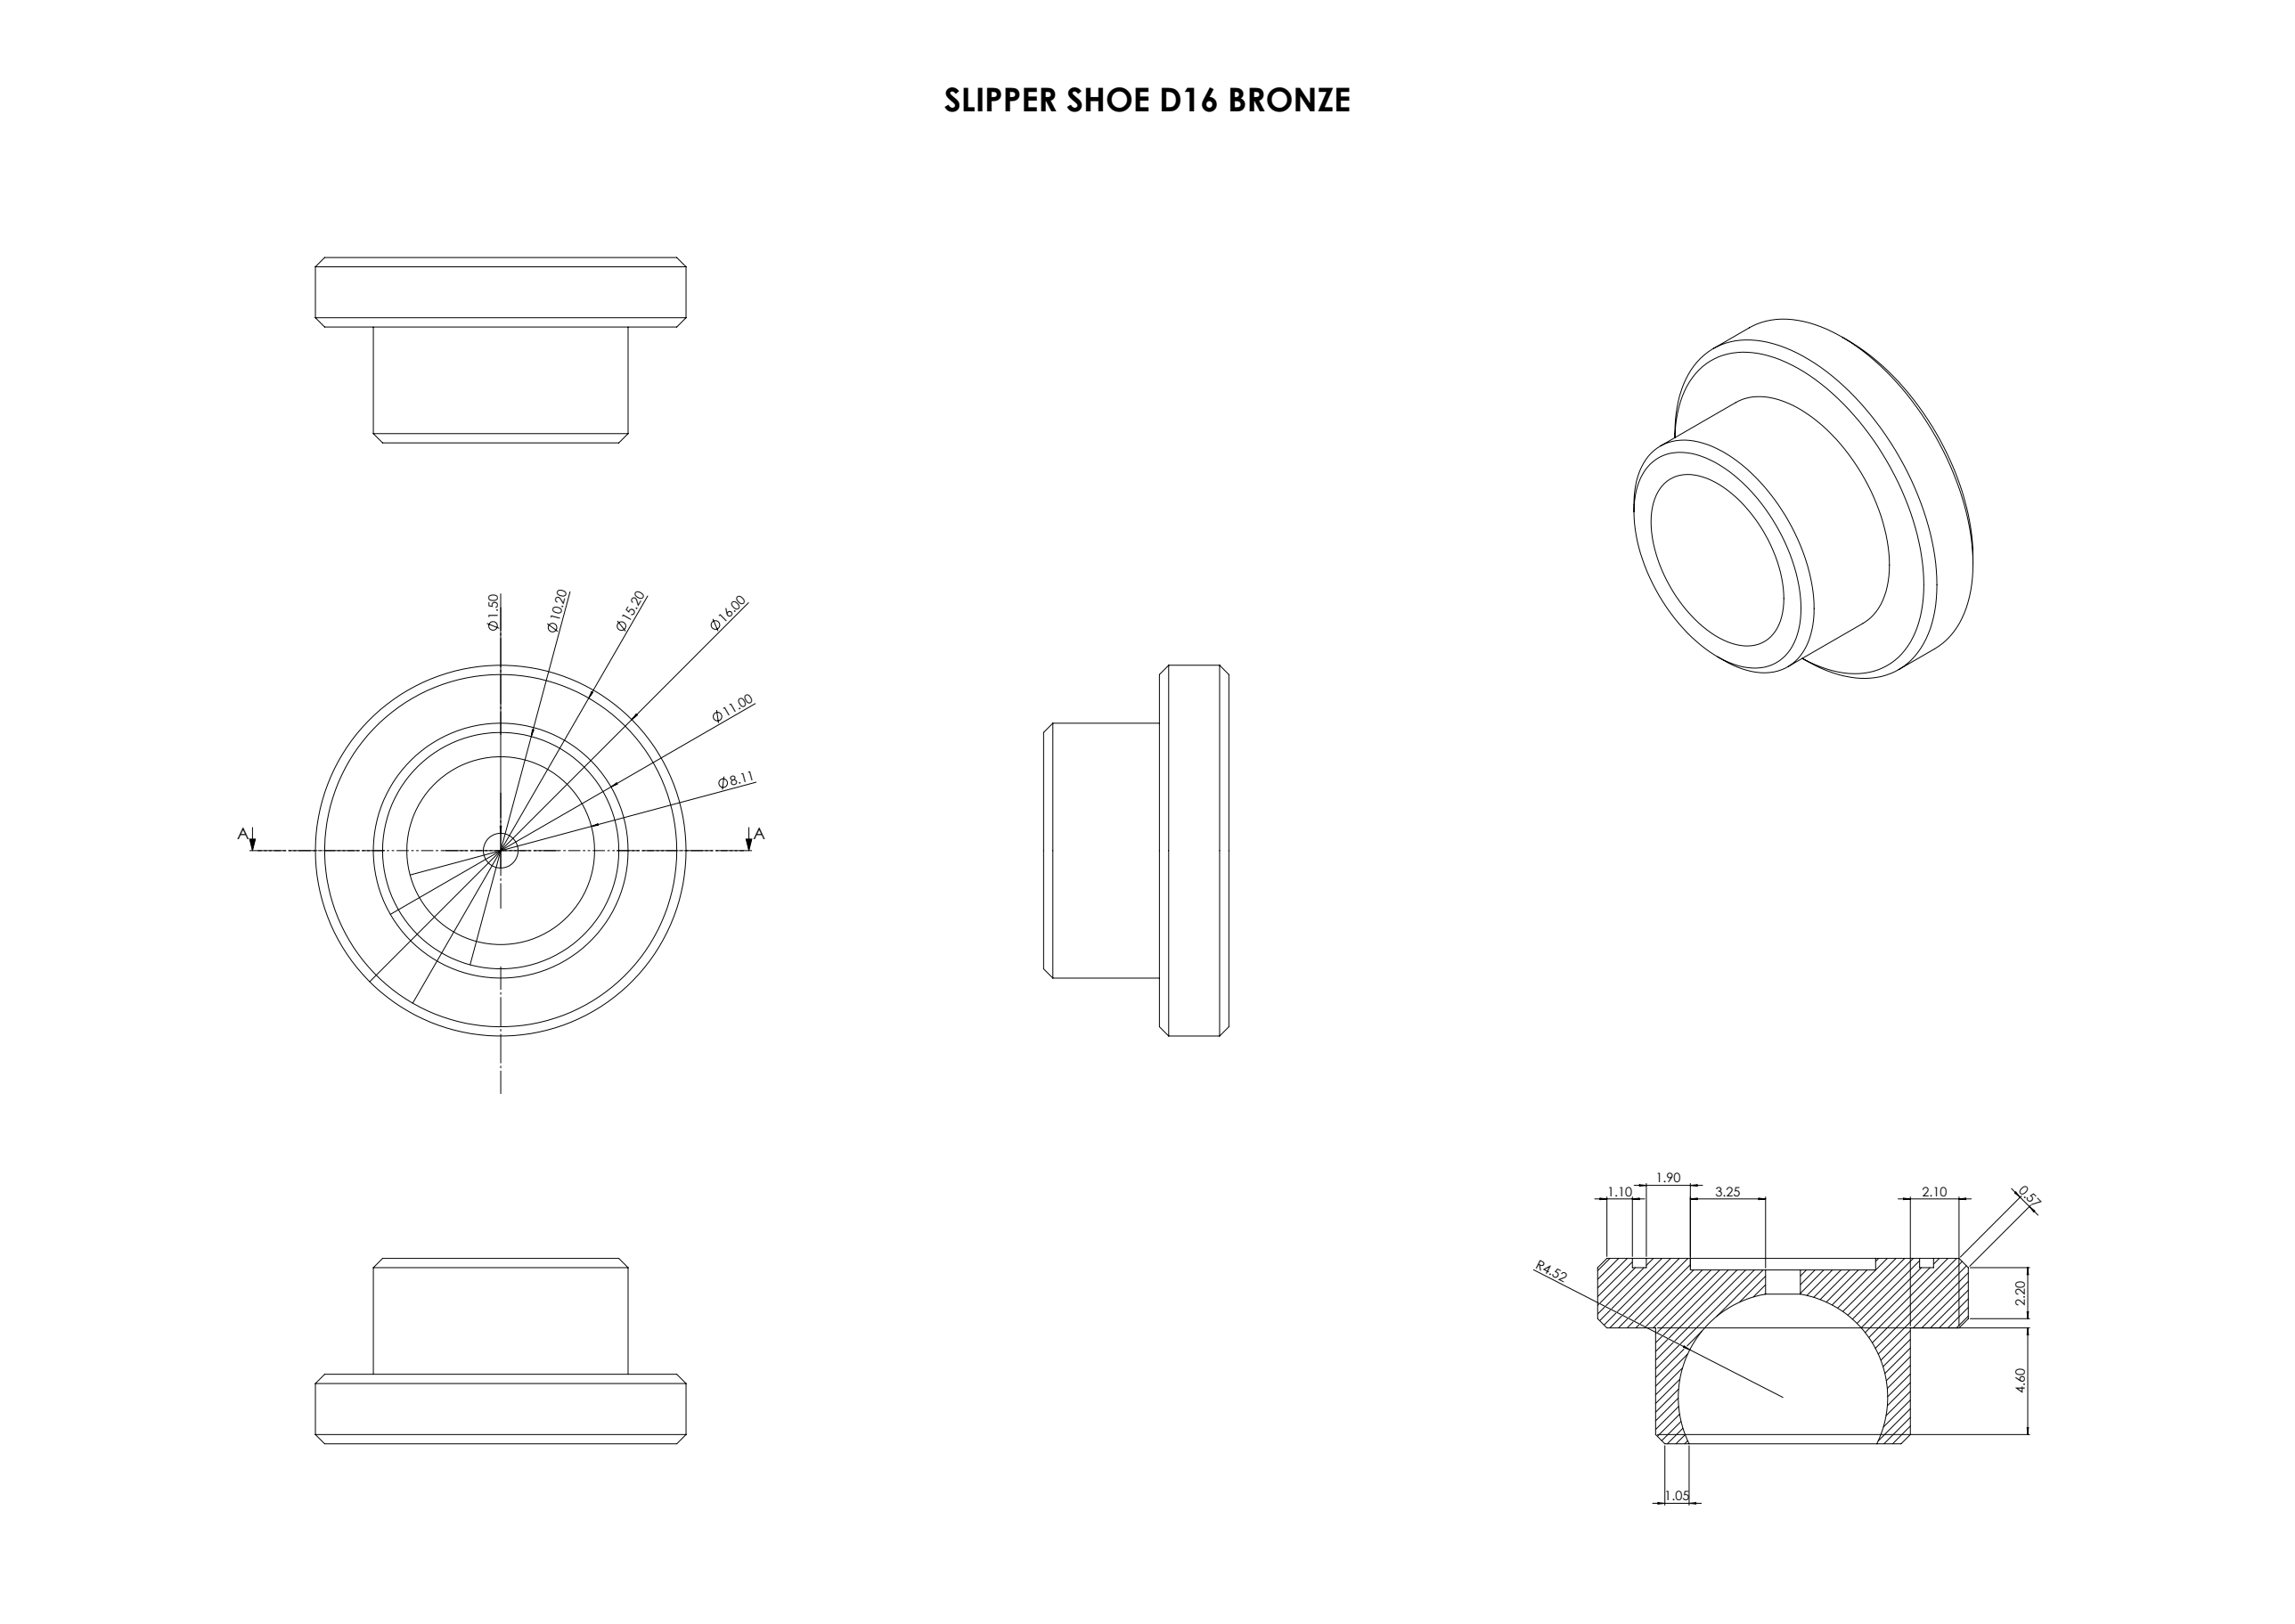
ISO-10303-21;
HEADER;
/* Generated by software containing ST-Developer
 * from STEP Tools, Inc. (www.steptools.com) 
 */

FILE_DESCRIPTION(
/* description */ (''),
/* implementation_level */ '2;1');

FILE_NAME(
/* name */ '07_Slipper_Shoe_D16_Bronze.step',
/* time_stamp */ '2026-10-23T00:52:27+05:00',
/* author */ (''),
/* organization */ (''),
/* preprocessor_version */ 'ST-DEVELOPER v20.2',
/* originating_system */ 'Autodesk Translation Framework v15.15.0.0',
/* authorisation */ '');

FILE_SCHEMA (('AUTOMOTIVE_DESIGN { 1 0 10303 214 3 1 1 }'));
ENDSEC;

DATA;
#10=MECHANICAL_DESIGN_GEOMETRIC_PRESENTATION_REPRESENTATION('',(#1569),#59204);
#1522=SHAPE_REPRESENTATION_RELATIONSHIP('SRR','None',#59311,#1542);
#1542=ADVANCED_BREP_SHAPE_REPRESENTATION('',(#1589),#59198);
#1569=STYLED_ITEM('',(#59600),#1589);
#1589=MANIFOLD_SOLID_BREP('Slipper',#22818);
#1598=SPHERICAL_SURFACE('',#24207,0.452);
#1752=FACE_BOUND('',#4994,.T.);
#1753=FACE_BOUND('',#4996,.T.);
#1754=FACE_BOUND('',#5000,.T.);
#1755=FACE_BOUND('',#5003,.T.);
#1756=FACE_BOUND('',#5008,.T.);
#1757=FACE_BOUND('',#5012,.T.);
#2152=PLANE('',#24204);
#2153=PLANE('',#24205);
#2154=PLANE('',#24213);
#2155=PLANE('',#24217);
#2156=PLANE('',#24224);
#2157=PLANE('',#24230);
#2573=CYLINDRICAL_SURFACE('',#24198,0.59);
#2574=CYLINDRICAL_SURFACE('',#24201,0.65);
#2575=CYLINDRICAL_SURFACE('',#24211,0.075);
#2576=CYLINDRICAL_SURFACE('',#24215,0.4);
#2577=CYLINDRICAL_SURFACE('',#24220,0.8);
#2578=CYLINDRICAL_SURFACE('',#24226,0.55);
#3533=FACE_OUTER_BOUND('',#4991,.T.);
#3534=FACE_OUTER_BOUND('',#4992,.T.);
#3535=FACE_OUTER_BOUND('',#4993,.T.);
#3536=FACE_OUTER_BOUND('',#4995,.T.);
#3537=FACE_OUTER_BOUND('',#4997,.T.);
#3538=FACE_OUTER_BOUND('',#4998,.T.);
#3539=FACE_OUTER_BOUND('',#4999,.T.);
#3540=FACE_OUTER_BOUND('',#5001,.T.);
#3541=FACE_OUTER_BOUND('',#5002,.T.);
#3542=FACE_OUTER_BOUND('',#5004,.T.);
#3543=FACE_OUTER_BOUND('',#5005,.T.);
#3544=FACE_OUTER_BOUND('',#5006,.T.);
#3545=FACE_OUTER_BOUND('',#5007,.T.);
#3546=FACE_OUTER_BOUND('',#5009,.T.);
#3547=FACE_OUTER_BOUND('',#5010,.T.);
#3548=FACE_OUTER_BOUND('',#5011,.T.);
#4991=EDGE_LOOP('',(#19016,#19017,#19018,#19019));
#4992=EDGE_LOOP('',(#19020,#19021,#19022,#19023));
#4993=EDGE_LOOP('',(#19024));
#4994=EDGE_LOOP('',(#19025));
#4995=EDGE_LOOP('',(#19026));
#4996=EDGE_LOOP('',(#19027));
#4997=EDGE_LOOP('',(#19028,#19029,#19030,#19031));
#4998=EDGE_LOOP('',(#19032,#19033,#19034,#19035));
#4999=EDGE_LOOP('',(#19036));
#5000=EDGE_LOOP('',(#19037));
#5001=EDGE_LOOP('',(#19038,#19039,#19040,#19041));
#5002=EDGE_LOOP('',(#19042));
#5003=EDGE_LOOP('',(#19043));
#5004=EDGE_LOOP('',(#19044,#19045,#19046,#19047));
#5005=EDGE_LOOP('',(#19048,#19049,#19050,#19051));
#5006=EDGE_LOOP('',(#19052,#19053,#19054,#19055));
#5007=EDGE_LOOP('',(#19056));
#5008=EDGE_LOOP('',(#19057));
#5009=EDGE_LOOP('',(#19058,#19059,#19060,#19061));
#5010=EDGE_LOOP('',(#19062,#19063,#19064,#19065));
#5011=EDGE_LOOP('',(#19066));
#5012=EDGE_LOOP('',(#19067));
#6501=LINE('',#47348,#7934);
#6502=LINE('',#47354,#7935);
#6503=LINE('',#47368,#7936);
#6504=LINE('',#47375,#7937);
#6505=LINE('',#47381,#7938);
#6506=LINE('',#47385,#7939);
#6507=LINE('',#47389,#7940);
#6508=LINE('',#47396,#7941);
#6509=LINE('',#47400,#7942);
#7934=VECTOR('',#28437,0.59);
#7935=VECTOR('',#28444,0.65);
#7936=VECTOR('',#28463,0.075);
#7937=VECTOR('',#28472,0.4);
#7938=VECTOR('',#28481,0.78);
#7939=VECTOR('',#28486,0.8);
#7940=VECTOR('',#28491,0.78);
#7941=VECTOR('',#28500,0.55);
#7942=VECTOR('',#28505,0.53);
#8874=CIRCLE('',#24199,0.59);
#8875=CIRCLE('',#24200,0.59);
#8876=CIRCLE('',#24202,0.65);
#8877=CIRCLE('',#24203,0.65);
#8878=CIRCLE('',#24206,0.76);
#8879=CIRCLE('',#24208,0.405344298097309);
#8880=CIRCLE('',#24209,0.452);
#8881=CIRCLE('',#24210,0.075);
#8882=CIRCLE('',#24212,0.075);
#8883=CIRCLE('',#24214,0.4);
#8884=CIRCLE('',#24216,0.4);
#8885=CIRCLE('',#24219,0.8);
#8886=CIRCLE('',#24221,0.8);
#8887=CIRCLE('',#24223,0.76);
#8888=CIRCLE('',#24225,0.55);
#8889=CIRCLE('',#24227,0.55);
#8890=CIRCLE('',#24229,0.51);
#10600=VERTEX_POINT('',#47345);
#10601=VERTEX_POINT('',#47347);
#10602=VERTEX_POINT('',#47351);
#10603=VERTEX_POINT('',#47353);
#10604=VERTEX_POINT('',#47358);
#10605=VERTEX_POINT('',#47361);
#10606=VERTEX_POINT('',#47363);
#10607=VERTEX_POINT('',#47367);
#10608=VERTEX_POINT('',#47371);
#10609=VERTEX_POINT('',#47374);
#10610=VERTEX_POINT('',#47379);
#10611=VERTEX_POINT('',#47383);
#10612=VERTEX_POINT('',#47387);
#10613=VERTEX_POINT('',#47391);
#10614=VERTEX_POINT('',#47394);
#10615=VERTEX_POINT('',#47398);
#13512=EDGE_CURVE('',#10600,#10600,#8874,.T.);
#13513=EDGE_CURVE('',#10600,#10601,#6501,.T.);
#13514=EDGE_CURVE('',#10601,#10601,#8875,.T.);
#13515=EDGE_CURVE('',#10602,#10602,#8876,.T.);
#13516=EDGE_CURVE('',#10602,#10603,#6502,.T.);
#13517=EDGE_CURVE('',#10603,#10603,#8877,.T.);
#13518=EDGE_CURVE('',#10604,#10604,#8878,.T.);
#13519=EDGE_CURVE('',#10605,#10605,#8879,.T.);
#13520=EDGE_CURVE('',#10605,#10606,#8880,.T.);
#13521=EDGE_CURVE('',#10606,#10606,#8881,.T.);
#13522=EDGE_CURVE('',#10606,#10607,#6503,.T.);
#13523=EDGE_CURVE('',#10607,#10607,#8882,.T.);
#13524=EDGE_CURVE('',#10608,#10608,#8883,.T.);
#13525=EDGE_CURVE('',#10608,#10609,#6504,.T.);
#13526=EDGE_CURVE('',#10609,#10609,#8884,.T.);
#13527=EDGE_CURVE('',#10610,#10610,#8885,.T.);
#13528=EDGE_CURVE('',#10610,#10604,#6505,.T.);
#13529=EDGE_CURVE('',#10611,#10611,#8886,.T.);
#13530=EDGE_CURVE('',#10611,#10610,#6506,.T.);
#13531=EDGE_CURVE('',#10612,#10612,#8887,.T.);
#13532=EDGE_CURVE('',#10612,#10611,#6507,.T.);
#13533=EDGE_CURVE('',#10613,#10613,#8888,.T.);
#13534=EDGE_CURVE('',#10614,#10614,#8889,.T.);
#13535=EDGE_CURVE('',#10614,#10613,#6508,.T.);
#13536=EDGE_CURVE('',#10615,#10615,#8890,.T.);
#13537=EDGE_CURVE('',#10615,#10614,#6509,.T.);
#19016=ORIENTED_EDGE('',*,*,#13512,.F.);
#19017=ORIENTED_EDGE('',*,*,#13513,.T.);
#19018=ORIENTED_EDGE('',*,*,#13514,.T.);
#19019=ORIENTED_EDGE('',*,*,#13513,.F.);
#19020=ORIENTED_EDGE('',*,*,#13515,.F.);
#19021=ORIENTED_EDGE('',*,*,#13516,.T.);
#19022=ORIENTED_EDGE('',*,*,#13517,.T.);
#19023=ORIENTED_EDGE('',*,*,#13516,.F.);
#19024=ORIENTED_EDGE('',*,*,#13517,.F.);
#19025=ORIENTED_EDGE('',*,*,#13514,.F.);
#19026=ORIENTED_EDGE('',*,*,#13518,.F.);
#19027=ORIENTED_EDGE('',*,*,#13515,.T.);
#19028=ORIENTED_EDGE('',*,*,#13519,.T.);
#19029=ORIENTED_EDGE('',*,*,#13520,.T.);
#19030=ORIENTED_EDGE('',*,*,#13521,.F.);
#19031=ORIENTED_EDGE('',*,*,#13520,.F.);
#19032=ORIENTED_EDGE('',*,*,#13521,.T.);
#19033=ORIENTED_EDGE('',*,*,#13522,.T.);
#19034=ORIENTED_EDGE('',*,*,#13523,.F.);
#19035=ORIENTED_EDGE('',*,*,#13522,.F.);
#19036=ORIENTED_EDGE('',*,*,#13524,.F.);
#19037=ORIENTED_EDGE('',*,*,#13523,.T.);
#19038=ORIENTED_EDGE('',*,*,#13524,.T.);
#19039=ORIENTED_EDGE('',*,*,#13525,.T.);
#19040=ORIENTED_EDGE('',*,*,#13526,.F.);
#19041=ORIENTED_EDGE('',*,*,#13525,.F.);
#19042=ORIENTED_EDGE('',*,*,#13512,.T.);
#19043=ORIENTED_EDGE('',*,*,#13526,.T.);
#19044=ORIENTED_EDGE('',*,*,#13527,.F.);
#19045=ORIENTED_EDGE('',*,*,#13528,.T.);
#19046=ORIENTED_EDGE('',*,*,#13518,.T.);
#19047=ORIENTED_EDGE('',*,*,#13528,.F.);
#19048=ORIENTED_EDGE('',*,*,#13529,.F.);
#19049=ORIENTED_EDGE('',*,*,#13530,.T.);
#19050=ORIENTED_EDGE('',*,*,#13527,.T.);
#19051=ORIENTED_EDGE('',*,*,#13530,.F.);
#19052=ORIENTED_EDGE('',*,*,#13531,.F.);
#19053=ORIENTED_EDGE('',*,*,#13532,.T.);
#19054=ORIENTED_EDGE('',*,*,#13529,.T.);
#19055=ORIENTED_EDGE('',*,*,#13532,.F.);
#19056=ORIENTED_EDGE('',*,*,#13531,.T.);
#19057=ORIENTED_EDGE('',*,*,#13533,.F.);
#19058=ORIENTED_EDGE('',*,*,#13534,.F.);
#19059=ORIENTED_EDGE('',*,*,#13535,.T.);
#19060=ORIENTED_EDGE('',*,*,#13533,.T.);
#19061=ORIENTED_EDGE('',*,*,#13535,.F.);
#19062=ORIENTED_EDGE('',*,*,#13536,.F.);
#19063=ORIENTED_EDGE('',*,*,#13537,.T.);
#19064=ORIENTED_EDGE('',*,*,#13534,.T.);
#19065=ORIENTED_EDGE('',*,*,#13537,.F.);
#19066=ORIENTED_EDGE('',*,*,#13536,.T.);
#19067=ORIENTED_EDGE('',*,*,#13519,.F.);
#21423=CONICAL_SURFACE('',#24218,0.78,0.785398163397448);
#21424=CONICAL_SURFACE('',#24222,0.78,0.785398163397449);
#21425=CONICAL_SURFACE('',#24228,0.53,0.785398163397449);
#22363=ADVANCED_FACE('',(#3533),#2573,.T.);
#22364=ADVANCED_FACE('',(#3534),#2574,.F.);
#22365=ADVANCED_FACE('',(#3535,#1752),#2152,.F.);
#22366=ADVANCED_FACE('',(#3536,#1753),#2153,.T.);
#22367=ADVANCED_FACE('',(#3537),#1598,.F.);
#22368=ADVANCED_FACE('',(#3538),#2575,.F.);
#22369=ADVANCED_FACE('',(#3539,#1754),#2154,.T.);
#22370=ADVANCED_FACE('',(#3540),#2576,.F.);
#22371=ADVANCED_FACE('',(#3541,#1755),#2155,.T.);
#22372=ADVANCED_FACE('',(#3542),#21423,.T.);
#22373=ADVANCED_FACE('',(#3543),#2577,.T.);
#22374=ADVANCED_FACE('',(#3544),#21424,.T.);
#22375=ADVANCED_FACE('',(#3545,#1756),#2156,.T.);
#22376=ADVANCED_FACE('',(#3546),#2578,.T.);
#22377=ADVANCED_FACE('',(#3547),#21425,.T.);
#22378=ADVANCED_FACE('',(#3548,#1757),#2157,.T.);
#22818=CLOSED_SHELL('',(#22363,#22364,#22365,#22366,#22367,#22368,#22369,
#22370,#22371,#22372,#22373,#22374,#22375,#22376,#22377,#22378));
#24197=AXIS2_PLACEMENT_3D('',#47343,#28431,#28432);
#24198=AXIS2_PLACEMENT_3D('',#47344,#28433,#28434);
#24199=AXIS2_PLACEMENT_3D('',#47346,#28435,#28436);
#24200=AXIS2_PLACEMENT_3D('',#47349,#28438,#28439);
#24201=AXIS2_PLACEMENT_3D('',#47350,#28440,#28441);
#24202=AXIS2_PLACEMENT_3D('',#47352,#28442,#28443);
#24203=AXIS2_PLACEMENT_3D('',#47355,#28445,#28446);
#24204=AXIS2_PLACEMENT_3D('',#47356,#28447,#28448);
#24205=AXIS2_PLACEMENT_3D('',#47357,#28449,#28450);
#24206=AXIS2_PLACEMENT_3D('',#47359,#28451,#28452);
#24207=AXIS2_PLACEMENT_3D('',#47360,#28453,#28454);
#24208=AXIS2_PLACEMENT_3D('',#47362,#28455,#28456);
#24209=AXIS2_PLACEMENT_3D('',#47364,#28457,#28458);
#24210=AXIS2_PLACEMENT_3D('',#47365,#28459,#28460);
#24211=AXIS2_PLACEMENT_3D('',#47366,#28461,#28462);
#24212=AXIS2_PLACEMENT_3D('',#47369,#28464,#28465);
#24213=AXIS2_PLACEMENT_3D('',#47370,#28466,#28467);
#24214=AXIS2_PLACEMENT_3D('',#47372,#28468,#28469);
#24215=AXIS2_PLACEMENT_3D('',#47373,#28470,#28471);
#24216=AXIS2_PLACEMENT_3D('',#47376,#28473,#28474);
#24217=AXIS2_PLACEMENT_3D('',#47377,#28475,#28476);
#24218=AXIS2_PLACEMENT_3D('',#47378,#28477,#28478);
#24219=AXIS2_PLACEMENT_3D('',#47380,#28479,#28480);
#24220=AXIS2_PLACEMENT_3D('',#47382,#28482,#28483);
#24221=AXIS2_PLACEMENT_3D('',#47384,#28484,#28485);
#24222=AXIS2_PLACEMENT_3D('',#47386,#28487,#28488);
#24223=AXIS2_PLACEMENT_3D('',#47388,#28489,#28490);
#24224=AXIS2_PLACEMENT_3D('',#47390,#28492,#28493);
#24225=AXIS2_PLACEMENT_3D('',#47392,#28494,#28495);
#24226=AXIS2_PLACEMENT_3D('',#47393,#28496,#28497);
#24227=AXIS2_PLACEMENT_3D('',#47395,#28498,#28499);
#24228=AXIS2_PLACEMENT_3D('',#47397,#28501,#28502);
#24229=AXIS2_PLACEMENT_3D('',#47399,#28503,#28504);
#24230=AXIS2_PLACEMENT_3D('',#47401,#28506,#28507);
#28431=DIRECTION('axis',(0.,0.,1.));
#28432=DIRECTION('refdir',(1.,0.,0.));
#28433=DIRECTION('center_axis',(0.,0.,1.));
#28434=DIRECTION('ref_axis',(1.,0.,0.));
#28435=DIRECTION('center_axis',(0.,0.,-1.));
#28436=DIRECTION('ref_axis',(1.,0.,0.));
#28437=DIRECTION('',(0.,0.,1.));
#28438=DIRECTION('center_axis',(0.,0.,-1.));
#28439=DIRECTION('ref_axis',(1.,0.,0.));
#28440=DIRECTION('center_axis',(0.,0.,1.));
#28441=DIRECTION('ref_axis',(1.,0.,0.));
#28442=DIRECTION('center_axis',(0.,0.,1.));
#28443=DIRECTION('ref_axis',(1.,0.,0.));
#28444=DIRECTION('',(0.,0.,1.));
#28445=DIRECTION('center_axis',(0.,0.,1.));
#28446=DIRECTION('ref_axis',(1.,0.,0.));
#28447=DIRECTION('center_axis',(0.,0.,1.));
#28448=DIRECTION('ref_axis',(1.,0.,0.));
#28449=DIRECTION('center_axis',(0.,0.,-1.));
#28450=DIRECTION('ref_axis',(-1.,0.,0.));
#28451=DIRECTION('center_axis',(0.,0.,1.));
#28452=DIRECTION('ref_axis',(1.,0.,0.));
#28453=DIRECTION('center_axis',(6.12323399573677E-17,0.,1.));
#28454=DIRECTION('ref_axis',(1.,0.,0.));
#28455=DIRECTION('center_axis',(0.,0.,1.));
#28456=DIRECTION('ref_axis',(1.,0.,0.));
#28457=DIRECTION('center_axis',(1.22464679914735E-16,-1.,0.));
#28458=DIRECTION('ref_axis',(-1.,-1.22464679914735E-16,0.));
#28459=DIRECTION('center_axis',(0.,0.,1.));
#28460=DIRECTION('ref_axis',(1.,0.,0.));
#28461=DIRECTION('center_axis',(0.,0.,1.));
#28462=DIRECTION('ref_axis',(1.,0.,0.));
#28463=DIRECTION('',(0.,0.,-1.));
#28464=DIRECTION('center_axis',(0.,0.,1.));
#28465=DIRECTION('ref_axis',(1.,0.,0.));
#28466=DIRECTION('center_axis',(0.,0.,-1.));
#28467=DIRECTION('ref_axis',(-1.,0.,0.));
#28468=DIRECTION('center_axis',(0.,0.,1.));
#28469=DIRECTION('ref_axis',(1.,0.,0.));
#28470=DIRECTION('center_axis',(0.,0.,1.));
#28471=DIRECTION('ref_axis',(1.,0.,0.));
#28472=DIRECTION('',(0.,0.,-1.));
#28473=DIRECTION('center_axis',(0.,0.,1.));
#28474=DIRECTION('ref_axis',(1.,0.,0.));
#28475=DIRECTION('center_axis',(0.,0.,-1.));
#28476=DIRECTION('ref_axis',(-1.,0.,0.));
#28477=DIRECTION('center_axis',(0.,0.,1.));
#28478=DIRECTION('ref_axis',(1.,0.,0.));
#28479=DIRECTION('center_axis',(0.,0.,1.));
#28480=DIRECTION('ref_axis',(1.,0.,0.));
#28481=DIRECTION('',(0.707106781186548,8.65956056235493E-17,-0.707106781186548));
#28482=DIRECTION('center_axis',(0.,0.,1.));
#28483=DIRECTION('ref_axis',(1.,0.,0.));
#28484=DIRECTION('center_axis',(0.,0.,1.));
#28485=DIRECTION('ref_axis',(1.,0.,0.));
#28486=DIRECTION('',(0.,0.,-1.));
#28487=DIRECTION('center_axis',(0.,0.,-1.));
#28488=DIRECTION('ref_axis',(1.,0.,0.));
#28489=DIRECTION('center_axis',(0.,0.,1.));
#28490=DIRECTION('ref_axis',(1.,0.,0.));
#28491=DIRECTION('',(-0.707106781186548,-8.65956056235494E-17,-0.707106781186547));
#28492=DIRECTION('center_axis',(0.,0.,1.));
#28493=DIRECTION('ref_axis',(1.,0.,0.));
#28494=DIRECTION('center_axis',(0.,0.,1.));
#28495=DIRECTION('ref_axis',(1.,0.,0.));
#28496=DIRECTION('center_axis',(0.,0.,1.));
#28497=DIRECTION('ref_axis',(1.,0.,0.));
#28498=DIRECTION('center_axis',(0.,0.,1.));
#28499=DIRECTION('ref_axis',(1.,0.,0.));
#28500=DIRECTION('',(0.,0.,-1.));
#28501=DIRECTION('center_axis',(0.,0.,-1.));
#28502=DIRECTION('ref_axis',(1.,0.,0.));
#28503=DIRECTION('center_axis',(0.,0.,1.));
#28504=DIRECTION('ref_axis',(1.,0.,0.));
#28505=DIRECTION('',(-0.707106781186548,-8.65956056235494E-17,-0.707106781186547));
#28506=DIRECTION('center_axis',(0.,0.,1.));
#28507=DIRECTION('ref_axis',(1.,0.,0.));
#47343=CARTESIAN_POINT('',(0.,0.,0.));
#47344=CARTESIAN_POINT('Origin',(0.,0.,-0.6));
#47345=CARTESIAN_POINT('',(-0.59,-7.22541611496939E-17,-0.6));
#47346=CARTESIAN_POINT('Origin',(0.,0.,-0.6));
#47347=CARTESIAN_POINT('',(-0.59,-7.22541611496939E-17,-0.56));
#47348=CARTESIAN_POINT('',(-0.59,-7.22541611496939E-17,-0.6));
#47349=CARTESIAN_POINT('Origin',(0.,0.,-0.56));
#47350=CARTESIAN_POINT('Origin',(0.,0.,-0.6));
#47351=CARTESIAN_POINT('',(-0.65,-7.9602041944578E-17,-0.6));
#47352=CARTESIAN_POINT('Origin',(0.,0.,-0.6));
#47353=CARTESIAN_POINT('',(-0.65,-7.9602041944578E-17,-0.56));
#47354=CARTESIAN_POINT('',(-0.65,-7.9602041944578E-17,-0.6));
#47355=CARTESIAN_POINT('Origin',(0.,0.,-0.56));
#47356=CARTESIAN_POINT('Origin',(0.,0.,-0.56));
#47357=CARTESIAN_POINT('Origin',(0.76,0.,-0.6));
#47358=CARTESIAN_POINT('',(-0.76,-9.30731567351988E-17,-0.6));
#47359=CARTESIAN_POINT('Origin',(0.,0.,-0.6));
#47360=CARTESIAN_POINT('Origin',(0.,0.,0.));
#47361=CARTESIAN_POINT('',(-0.405344298097309,-4.964035972175E-17,0.2));
#47362=CARTESIAN_POINT('Origin',(0.,0.,0.2));
#47363=CARTESIAN_POINT('',(-0.075,-9.18485099360515E-18,-0.445734225744445));
#47364=CARTESIAN_POINT('Origin',(0.,0.,0.));
#47365=CARTESIAN_POINT('Origin',(0.,0.,-0.445734225744445));
#47366=CARTESIAN_POINT('Origin',(0.,0.,-0.497867112872223));
#47367=CARTESIAN_POINT('',(-0.075,-9.18485099360515E-18,-0.55));
#47368=CARTESIAN_POINT('',(-0.075,-9.18485099360515E-18,-0.497867112872223));
#47369=CARTESIAN_POINT('Origin',(0.,0.,-0.55));
#47370=CARTESIAN_POINT('Origin',(0.4,0.,-0.55));
#47371=CARTESIAN_POINT('',(-0.4,-4.89858719658941E-17,-0.55));
#47372=CARTESIAN_POINT('Origin',(0.,0.,-0.55));
#47373=CARTESIAN_POINT('Origin',(0.,0.,-0.575));
#47374=CARTESIAN_POINT('',(-0.4,-4.89858719658941E-17,-0.6));
#47375=CARTESIAN_POINT('',(-0.4,-4.89858719658941E-17,-0.575));
#47376=CARTESIAN_POINT('Origin',(0.,0.,-0.6));
#47377=CARTESIAN_POINT('Origin',(0.76,0.,-0.6));
#47378=CARTESIAN_POINT('Origin',(0.,0.,-0.58));
#47379=CARTESIAN_POINT('',(-0.8,-9.79717439317883E-17,-0.56));
#47380=CARTESIAN_POINT('Origin',(0.,0.,-0.56));
#47381=CARTESIAN_POINT('',(-0.78,-9.55224503334935E-17,-0.58));
#47382=CARTESIAN_POINT('Origin',(0.,0.,-0.45));
#47383=CARTESIAN_POINT('',(-0.8,-9.79717439317883E-17,-0.34));
#47384=CARTESIAN_POINT('Origin',(0.,0.,-0.34));
#47385=CARTESIAN_POINT('',(-0.8,-9.79717439317883E-17,-0.45));
#47386=CARTESIAN_POINT('Origin',(0.,0.,-0.32));
#47387=CARTESIAN_POINT('',(-0.76,-9.30731567351988E-17,-0.3));
#47388=CARTESIAN_POINT('Origin',(0.,0.,-0.3));
#47389=CARTESIAN_POINT('',(-0.78,-9.55224503334935E-17,-0.32));
#47390=CARTESIAN_POINT('Origin',(0.55,0.,-0.3));
#47391=CARTESIAN_POINT('',(-0.55,-6.73555739531044E-17,-0.3));
#47392=CARTESIAN_POINT('Origin',(0.,0.,-0.3));
#47393=CARTESIAN_POINT('Origin',(0.,0.,-0.07));
#47394=CARTESIAN_POINT('',(-0.55,-6.73555739531044E-17,0.16));
#47395=CARTESIAN_POINT('Origin',(0.,0.,0.16));
#47396=CARTESIAN_POINT('',(-0.55,-6.73555739531044E-17,-0.07));
#47397=CARTESIAN_POINT('Origin',(0.,0.,0.18));
#47398=CARTESIAN_POINT('',(-0.51,-6.2456986756515E-17,0.2));
#47399=CARTESIAN_POINT('Origin',(0.,0.,0.2));
#47400=CARTESIAN_POINT('',(-0.53,-6.49062803548097E-17,0.18));
#47401=CARTESIAN_POINT('Origin',(0.405344298097309,0.,0.2));
#59176=UNCERTAINTY_MEASURE_WITH_UNIT(LENGTH_MEASURE(0.001),#59205,
'DISTANCE_ACCURACY_VALUE',
'Maximum model space distance between geometric entities at asserted c
onnectivities');
#59182=UNCERTAINTY_MEASURE_WITH_UNIT(LENGTH_MEASURE(0.001),#59205,
'DISTANCE_ACCURACY_VALUE',
'Maximum model space distance between geometric entities at asserted c
onnectivities');
#59198=(
GEOMETRIC_REPRESENTATION_CONTEXT(3)
GLOBAL_UNCERTAINTY_ASSIGNED_CONTEXT((#59176))
GLOBAL_UNIT_ASSIGNED_CONTEXT((#59205,#59207,#59208))
REPRESENTATION_CONTEXT('','3D')
);
#59204=(
GEOMETRIC_REPRESENTATION_CONTEXT(3)
GLOBAL_UNCERTAINTY_ASSIGNED_CONTEXT((#59182))
GLOBAL_UNIT_ASSIGNED_CONTEXT((#59205,#59207,#59208))
REPRESENTATION_CONTEXT('','3D')
);
#59205=(
LENGTH_UNIT()
NAMED_UNIT(*)
SI_UNIT(.CENTI.,.METRE.)
);
#59207=(
NAMED_UNIT(*)
PLANE_ANGLE_UNIT()
SI_UNIT($,.RADIAN.)
);
#59208=(
NAMED_UNIT(*)
SI_UNIT($,.STERADIAN.)
SOLID_ANGLE_UNIT()
);
#59224=SHAPE_DEFINITION_REPRESENTATION(#59245,#59311);
#59245=PRODUCT_DEFINITION_SHAPE('',$,#59333);
#59311=SHAPE_REPRESENTATION('',(#24197),#59198);
#59317=PRODUCT_DEFINITION_CONTEXT('part definition',#59382,'design');
#59333=PRODUCT_DEFINITION('2026-10-23-00-47-18-058',
'07_Slipper_Shoe_D16_Bronze',#59354,#59317);
#59354=PRODUCT_DEFINITION_FORMATION('',$,#59399);
#59382=APPLICATION_CONTEXT(
'Core Data for Automotive Mechanical Design Process');
#59383=PRODUCT_CONTEXT('part definition',#59382,'mechanical');
#59399=PRODUCT('2026-10-23-00-47-18-058','07_Slipper_Shoe_D16_Bronze',$,
(#59383));
#59594=COLOUR_RGB('Off White',0.89,0.88,0.83);
#59595=FILL_AREA_STYLE_COLOUR('',#59594);
#59596=FILL_AREA_STYLE('',(#59595));
#59597=SURFACE_STYLE_FILL_AREA(#59596);
#59598=SURFACE_SIDE_STYLE('',(#59597));
#59599=SURFACE_STYLE_USAGE(.BOTH.,#59598);
#59600=PRESENTATION_STYLE_ASSIGNMENT((#59599));
ENDSEC;
END-ISO-10303-21;
